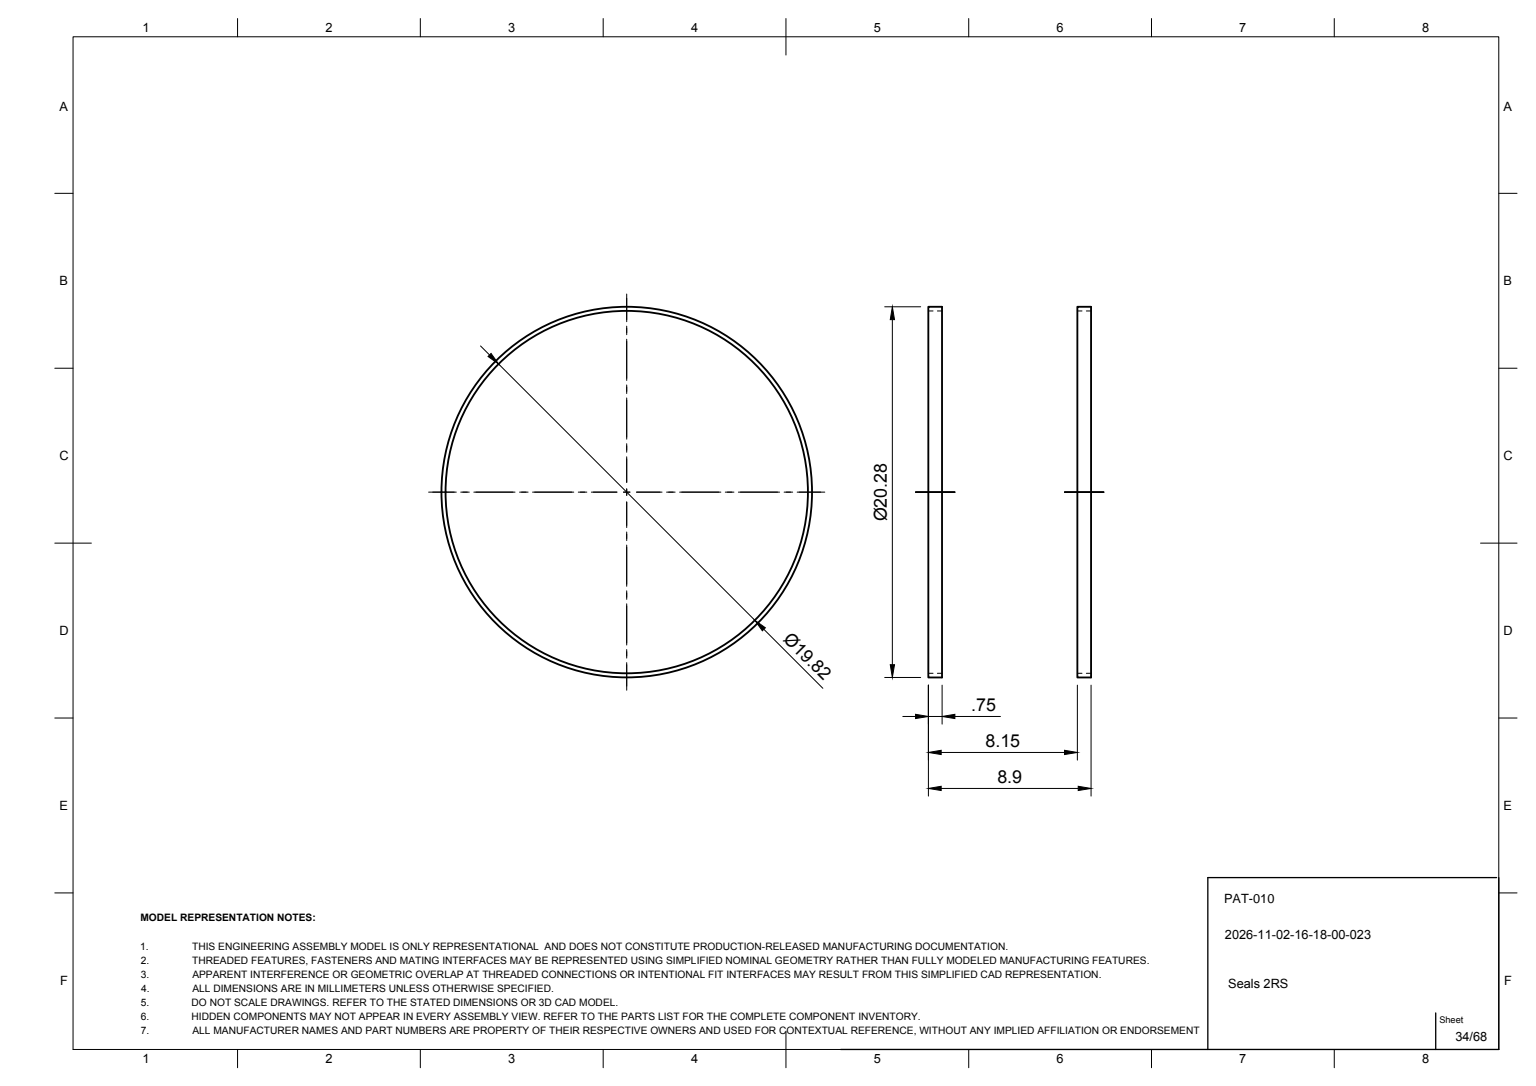
ISO-10303-21;
HEADER;
/* Generated by software containing ST-Developer
 * from STEP Tools, Inc. (www.steptools.com) 
 */

FILE_DESCRIPTION(
/* description */ ('Belt conveyor head drive unit'),
/* implementation_level */ '2;1');

FILE_NAME(
/* name */ 'Seals 2RS.step',
/* time_stamp */ '2026-10-28T03:26:19-07:00',
/* author */ (''),
/* organization */ (''),
/* preprocessor_version */ 'ST-DEVELOPER v20.2',
/* originating_system */ 'Autodesk Translation Framework v15.17.0.0',
/* authorisation */ '');

FILE_SCHEMA (('AUTOMOTIVE_DESIGN { 1 0 10303 214 3 1 1 }'));
ENDSEC;

DATA;
#10=MECHANICAL_DESIGN_GEOMETRIC_PRESENTATION_REPRESENTATION('',(#885,#886),#27069);
#740=SHAPE_REPRESENTATION_RELATIONSHIP('SRR','None',#27385,#809);
#809=ADVANCED_BREP_SHAPE_REPRESENTATION('',(#970,#971),#27027);
#885=STYLED_ITEM('',(#27797),#970);
#886=STYLED_ITEM('',(#27797),#971);
#970=MANIFOLD_SOLID_BREP('Body1',#13750);
#971=MANIFOLD_SOLID_BREP('Body2',#13751);
#1156=FACE_BOUND('',#2923,.T.);
#1157=FACE_BOUND('',#2926,.T.);
#1158=FACE_BOUND('',#2929,.T.);
#1159=FACE_BOUND('',#2932,.T.);
#1450=PLANE('',#15302);
#1451=PLANE('',#15307);
#1452=PLANE('',#15310);
#1453=PLANE('',#15315);
#1978=FACE_OUTER_BOUND('',#2922,.T.);
#1979=FACE_OUTER_BOUND('',#2924,.T.);
#1980=FACE_OUTER_BOUND('',#2925,.T.);
#1981=FACE_OUTER_BOUND('',#2927,.T.);
#1982=FACE_OUTER_BOUND('',#2928,.T.);
#1983=FACE_OUTER_BOUND('',#2930,.T.);
#1984=FACE_OUTER_BOUND('',#2931,.T.);
#1985=FACE_OUTER_BOUND('',#2933,.T.);
#2922=EDGE_LOOP('',(#10460));
#2923=EDGE_LOOP('',(#10461));
#2924=EDGE_LOOP('',(#10462,#10463,#10464,#10465));
#2925=EDGE_LOOP('',(#10466));
#2926=EDGE_LOOP('',(#10467));
#2927=EDGE_LOOP('',(#10468,#10469,#10470,#10471));
#2928=EDGE_LOOP('',(#10472));
#2929=EDGE_LOOP('',(#10473));
#2930=EDGE_LOOP('',(#10474,#10475,#10476,#10477));
#2931=EDGE_LOOP('',(#10478));
#2932=EDGE_LOOP('',(#10479));
#2933=EDGE_LOOP('',(#10480,#10481,#10482,#10483));
#3871=LINE('',#22957,#4663);
#3872=LINE('',#22962,#4664);
#3873=LINE('',#22971,#4665);
#3874=LINE('',#22976,#4666);
#4663=VECTOR('',#18297,1.013815);
#4664=VECTOR('',#18304,0.991185);
#4665=VECTOR('',#18315,1.013815);
#4666=VECTOR('',#18322,0.991185);
#5442=CIRCLE('',#15303,1.013815);
#5443=CIRCLE('',#15304,0.991185);
#5444=CIRCLE('',#15306,1.013815);
#5445=CIRCLE('',#15308,0.991185);
#5446=CIRCLE('',#15311,1.013815);
#5447=CIRCLE('',#15312,0.991185);
#5448=CIRCLE('',#15314,1.013815);
#5449=CIRCLE('',#15316,0.991185);
#6463=VERTEX_POINT('',#22950);
#6464=VERTEX_POINT('',#22952);
#6465=VERTEX_POINT('',#22955);
#6466=VERTEX_POINT('',#22959);
#6467=VERTEX_POINT('',#22964);
#6468=VERTEX_POINT('',#22966);
#6469=VERTEX_POINT('',#22969);
#6470=VERTEX_POINT('',#22973);
#7922=EDGE_CURVE('',#6463,#6463,#5442,.T.);
#7923=EDGE_CURVE('',#6464,#6464,#5443,.T.);
#7924=EDGE_CURVE('',#6465,#6465,#5444,.T.);
#7925=EDGE_CURVE('',#6465,#6463,#3871,.T.);
#7926=EDGE_CURVE('',#6466,#6466,#5445,.T.);
#7927=EDGE_CURVE('',#6466,#6464,#3872,.T.);
#7928=EDGE_CURVE('',#6467,#6467,#5446,.T.);
#7929=EDGE_CURVE('',#6468,#6468,#5447,.T.);
#7930=EDGE_CURVE('',#6469,#6469,#5448,.T.);
#7931=EDGE_CURVE('',#6469,#6467,#3873,.T.);
#7932=EDGE_CURVE('',#6470,#6470,#5449,.T.);
#7933=EDGE_CURVE('',#6470,#6468,#3874,.T.);
#10460=ORIENTED_EDGE('',*,*,#7922,.F.);
#10461=ORIENTED_EDGE('',*,*,#7923,.T.);
#10462=ORIENTED_EDGE('',*,*,#7924,.F.);
#10463=ORIENTED_EDGE('',*,*,#7925,.T.);
#10464=ORIENTED_EDGE('',*,*,#7922,.T.);
#10465=ORIENTED_EDGE('',*,*,#7925,.F.);
#10466=ORIENTED_EDGE('',*,*,#7924,.T.);
#10467=ORIENTED_EDGE('',*,*,#7926,.F.);
#10468=ORIENTED_EDGE('',*,*,#7926,.T.);
#10469=ORIENTED_EDGE('',*,*,#7927,.T.);
#10470=ORIENTED_EDGE('',*,*,#7923,.F.);
#10471=ORIENTED_EDGE('',*,*,#7927,.F.);
#10472=ORIENTED_EDGE('',*,*,#7928,.F.);
#10473=ORIENTED_EDGE('',*,*,#7929,.T.);
#10474=ORIENTED_EDGE('',*,*,#7930,.F.);
#10475=ORIENTED_EDGE('',*,*,#7931,.T.);
#10476=ORIENTED_EDGE('',*,*,#7928,.T.);
#10477=ORIENTED_EDGE('',*,*,#7931,.F.);
#10478=ORIENTED_EDGE('',*,*,#7930,.T.);
#10479=ORIENTED_EDGE('',*,*,#7932,.F.);
#10480=ORIENTED_EDGE('',*,*,#7932,.T.);
#10481=ORIENTED_EDGE('',*,*,#7933,.T.);
#10482=ORIENTED_EDGE('',*,*,#7929,.F.);
#10483=ORIENTED_EDGE('',*,*,#7933,.F.);
#12682=CYLINDRICAL_SURFACE('',#15305,1.013815);
#12683=CYLINDRICAL_SURFACE('',#15309,0.991185);
#12684=CYLINDRICAL_SURFACE('',#15313,1.013815);
#12685=CYLINDRICAL_SURFACE('',#15317,0.991185);
#13257=ADVANCED_FACE('',(#1978,#1156),#1450,.T.);
#13258=ADVANCED_FACE('',(#1979),#12682,.T.);
#13259=ADVANCED_FACE('',(#1980,#1157),#1451,.T.);
#13260=ADVANCED_FACE('',(#1981),#12683,.F.);
#13261=ADVANCED_FACE('',(#1982,#1158),#1452,.T.);
#13262=ADVANCED_FACE('',(#1983),#12684,.T.);
#13263=ADVANCED_FACE('',(#1984,#1159),#1453,.T.);
#13264=ADVANCED_FACE('',(#1985),#12685,.F.);
#13750=CLOSED_SHELL('',(#13257,#13258,#13259,#13260));
#13751=CLOSED_SHELL('',(#13261,#13262,#13263,#13264));
#15301=AXIS2_PLACEMENT_3D('',#22948,#18285,#18286);
#15302=AXIS2_PLACEMENT_3D('',#22949,#18287,#18288);
#15303=AXIS2_PLACEMENT_3D('',#22951,#18289,#18290);
#15304=AXIS2_PLACEMENT_3D('',#22953,#18291,#18292);
#15305=AXIS2_PLACEMENT_3D('',#22954,#18293,#18294);
#15306=AXIS2_PLACEMENT_3D('',#22956,#18295,#18296);
#15307=AXIS2_PLACEMENT_3D('',#22958,#18298,#18299);
#15308=AXIS2_PLACEMENT_3D('',#22960,#18300,#18301);
#15309=AXIS2_PLACEMENT_3D('',#22961,#18302,#18303);
#15310=AXIS2_PLACEMENT_3D('',#22963,#18305,#18306);
#15311=AXIS2_PLACEMENT_3D('',#22965,#18307,#18308);
#15312=AXIS2_PLACEMENT_3D('',#22967,#18309,#18310);
#15313=AXIS2_PLACEMENT_3D('',#22968,#18311,#18312);
#15314=AXIS2_PLACEMENT_3D('',#22970,#18313,#18314);
#15315=AXIS2_PLACEMENT_3D('',#22972,#18316,#18317);
#15316=AXIS2_PLACEMENT_3D('',#22974,#18318,#18319);
#15317=AXIS2_PLACEMENT_3D('',#22975,#18320,#18321);
#18285=DIRECTION('axis',(0.,0.,1.));
#18286=DIRECTION('refdir',(1.,0.,0.));
#18287=DIRECTION('center_axis',(0.,1.,0.));
#18288=DIRECTION('ref_axis',(0.,0.,1.));
#18289=DIRECTION('center_axis',(0.,-1.,0.));
#18290=DIRECTION('ref_axis',(1.,0.,0.));
#18291=DIRECTION('center_axis',(0.,-1.,0.));
#18292=DIRECTION('ref_axis',(1.,0.,0.));
#18293=DIRECTION('center_axis',(0.,-1.,0.));
#18294=DIRECTION('ref_axis',(1.,0.,0.));
#18295=DIRECTION('center_axis',(0.,-1.,0.));
#18296=DIRECTION('ref_axis',(1.,0.,0.));
#18297=DIRECTION('',(0.,1.,0.));
#18298=DIRECTION('center_axis',(0.,-1.,0.));
#18299=DIRECTION('ref_axis',(0.,0.,-1.));
#18300=DIRECTION('center_axis',(0.,-1.,0.));
#18301=DIRECTION('ref_axis',(1.,0.,0.));
#18302=DIRECTION('center_axis',(0.,-1.,0.));
#18303=DIRECTION('ref_axis',(1.,0.,0.));
#18304=DIRECTION('',(0.,1.,0.));
#18305=DIRECTION('center_axis',(0.,1.,0.));
#18306=DIRECTION('ref_axis',(0.,0.,1.));
#18307=DIRECTION('center_axis',(0.,-1.,0.));
#18308=DIRECTION('ref_axis',(1.,0.,0.));
#18309=DIRECTION('center_axis',(0.,-1.,0.));
#18310=DIRECTION('ref_axis',(1.,0.,0.));
#18311=DIRECTION('center_axis',(0.,-1.,0.));
#18312=DIRECTION('ref_axis',(1.,0.,0.));
#18313=DIRECTION('center_axis',(0.,-1.,0.));
#18314=DIRECTION('ref_axis',(1.,0.,0.));
#18315=DIRECTION('',(0.,1.,0.));
#18316=DIRECTION('center_axis',(0.,-1.,0.));
#18317=DIRECTION('ref_axis',(0.,0.,-1.));
#18318=DIRECTION('center_axis',(0.,-1.,0.));
#18319=DIRECTION('ref_axis',(1.,0.,0.));
#18320=DIRECTION('center_axis',(0.,-1.,0.));
#18321=DIRECTION('ref_axis',(1.,0.,0.));
#18322=DIRECTION('',(0.,1.,0.));
#22948=CARTESIAN_POINT('',(0.,0.,0.));
#22949=CARTESIAN_POINT('Origin',(1.013815,0.445,0.));
#22950=CARTESIAN_POINT('',(-1.013815,0.445,-1.24156529467757E-16));
#22951=CARTESIAN_POINT('Origin',(0.,0.445,0.));
#22952=CARTESIAN_POINT('',(-0.991185,0.445,-1.21385153761287E-16));
#22953=CARTESIAN_POINT('Origin',(0.,0.445,0.));
#22954=CARTESIAN_POINT('Origin',(0.,0.4075,0.));
#22955=CARTESIAN_POINT('',(-1.013815,0.37,-1.24156529467757E-16));
#22956=CARTESIAN_POINT('Origin',(0.,0.37,0.));
#22957=CARTESIAN_POINT('',(-1.013815,0.4075,-1.24156529467757E-16));
#22958=CARTESIAN_POINT('Origin',(0.991185,0.37,0.));
#22959=CARTESIAN_POINT('',(-0.991185,0.37,-1.21385153761287E-16));
#22960=CARTESIAN_POINT('Origin',(0.,0.37,0.));
#22961=CARTESIAN_POINT('Origin',(0.,0.4075,0.));
#22962=CARTESIAN_POINT('',(-0.991185,0.4075,-1.21385153761287E-16));
#22963=CARTESIAN_POINT('Origin',(1.013815,-0.37,0.));
#22964=CARTESIAN_POINT('',(-1.013815,-0.37,-1.24156529467757E-16));
#22965=CARTESIAN_POINT('Origin',(0.,-0.37,0.));
#22966=CARTESIAN_POINT('',(-0.991185,-0.37,-1.21385153761287E-16));
#22967=CARTESIAN_POINT('Origin',(0.,-0.37,0.));
#22968=CARTESIAN_POINT('Origin',(0.,-0.4075,0.));
#22969=CARTESIAN_POINT('',(-1.013815,-0.445,-1.24156529467757E-16));
#22970=CARTESIAN_POINT('Origin',(0.,-0.445,0.));
#22971=CARTESIAN_POINT('',(-1.013815,-0.4075,-1.24156529467757E-16));
#22972=CARTESIAN_POINT('Origin',(0.991185,-0.445,0.));
#22973=CARTESIAN_POINT('',(-0.991185,-0.445,-1.21385153761287E-16));
#22974=CARTESIAN_POINT('Origin',(0.,-0.445,0.));
#22975=CARTESIAN_POINT('Origin',(0.,-0.4075,0.));
#22976=CARTESIAN_POINT('',(-0.991185,-0.4075,-1.21385153761287E-16));
#26950=UNCERTAINTY_MEASURE_WITH_UNIT(LENGTH_MEASURE(0.001),#27070,
'DISTANCE_ACCURACY_VALUE',
'Maximum model space distance between geometric entities at asserted c
onnectivities');
#26992=UNCERTAINTY_MEASURE_WITH_UNIT(LENGTH_MEASURE(0.001),#27070,
'DISTANCE_ACCURACY_VALUE',
'Maximum model space distance between geometric entities at asserted c
onnectivities');
#27027=(
GEOMETRIC_REPRESENTATION_CONTEXT(3)
GLOBAL_UNCERTAINTY_ASSIGNED_CONTEXT((#26950))
GLOBAL_UNIT_ASSIGNED_CONTEXT((#27070,#27072,#27073))
REPRESENTATION_CONTEXT('','3D')
);
#27069=(
GEOMETRIC_REPRESENTATION_CONTEXT(3)
GLOBAL_UNCERTAINTY_ASSIGNED_CONTEXT((#26992))
GLOBAL_UNIT_ASSIGNED_CONTEXT((#27070,#27072,#27073))
REPRESENTATION_CONTEXT('','3D')
);
#27070=(
LENGTH_UNIT()
NAMED_UNIT(*)
SI_UNIT(.CENTI.,.METRE.)
);
#27072=(
NAMED_UNIT(*)
PLANE_ANGLE_UNIT()
SI_UNIT($,.RADIAN.)
);
#27073=(
NAMED_UNIT(*)
SI_UNIT($,.STERADIAN.)
SOLID_ANGLE_UNIT()
);
#27108=SHAPE_DEFINITION_REPRESENTATION(#27184,#27385);
#27184=PRODUCT_DEFINITION_SHAPE('',$,#27462);
#27385=SHAPE_REPRESENTATION('',(#15301),#27027);
#27427=PRODUCT_DEFINITION_CONTEXT('part definition',#27657,'design');
#27462=PRODUCT_DEFINITION('Seals 2RS','Seals 2RS',#27538,#27427);
#27538=PRODUCT_DEFINITION_FORMATION('',$,#27693);
#27657=APPLICATION_CONTEXT(
'Core Data for Automotive Mechanical Design Process');
#27658=PRODUCT_CONTEXT('part definition',#27657,'mechanical');
#27693=PRODUCT('Seals 2RS','Seals 2RS','Seals 2RS',(#27658));
#27791=COLOUR_RGB('Grey',0.48,0.52,0.57);
#27792=FILL_AREA_STYLE_COLOUR('',#27791);
#27793=FILL_AREA_STYLE('',(#27792));
#27794=SURFACE_STYLE_FILL_AREA(#27793);
#27795=SURFACE_SIDE_STYLE('',(#27794));
#27796=SURFACE_STYLE_USAGE(.BOTH.,#27795);
#27797=PRESENTATION_STYLE_ASSIGNMENT((#27796));
ENDSEC;
END-ISO-10303-21;
